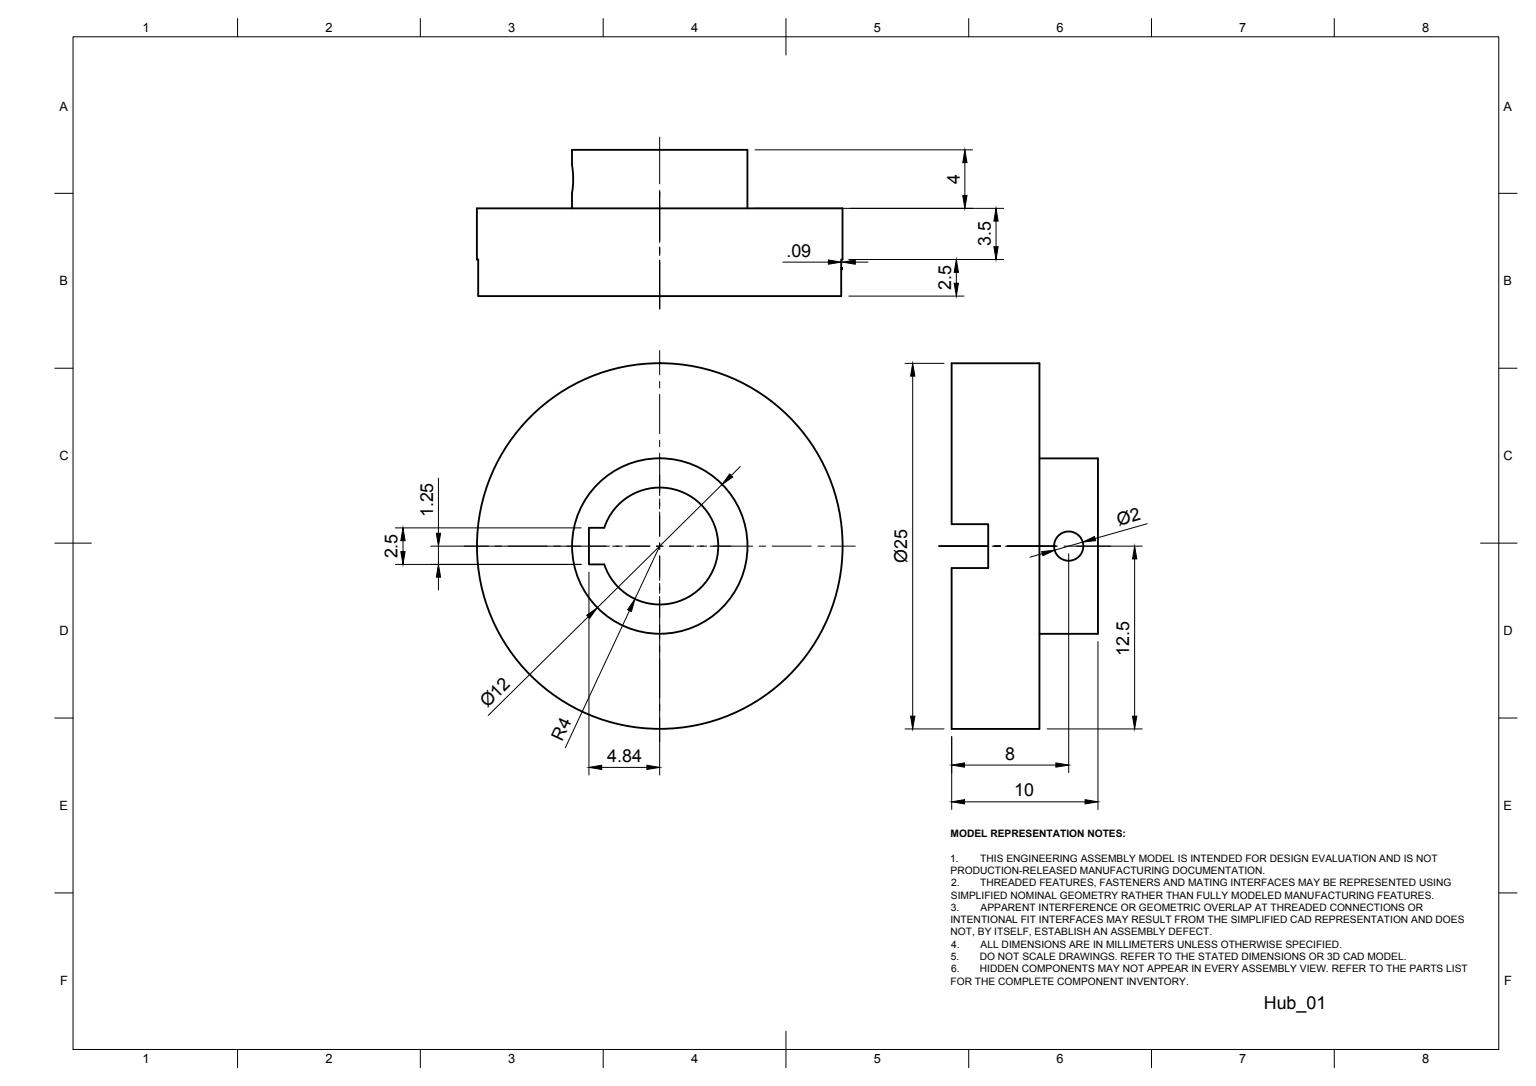
ISO-10303-21;
HEADER;
/* Generated by software containing ST-Developer
 * from STEP Tools, Inc. (www.steptools.com) 
 */

FILE_DESCRIPTION(
/* description */ (''),
/* implementation_level */ '2;1');

FILE_NAME(
/* name */ 'Hub_01.step',
/* time_stamp */ '2026-10-05T22:24:12-07:00',
/* author */ (''),
/* organization */ (''),
/* preprocessor_version */ 'ST-DEVELOPER v20.2',
/* originating_system */ 'Autodesk Translation Framework v15.15.0.0',
/* authorisation */ '');

FILE_SCHEMA (('AUTOMOTIVE_DESIGN { 1 0 10303 214 3 1 1 }'));
ENDSEC;

DATA;
#10=MECHANICAL_DESIGN_GEOMETRIC_PRESENTATION_REPRESENTATION('',(#53),#2116);
#39=SHAPE_REPRESENTATION_RELATIONSHIP('SRR','None',#2145,#46);
#46=ADVANCED_BREP_SHAPE_REPRESENTATION('',(#60),#2109);
#53=STYLED_ITEM('',(#2189),#60);
#60=MANIFOLD_SOLID_BREP('Body1',#1147);
#67=FACE_BOUND('',#201,.T.);
#68=FACE_BOUND('',#211,.T.);
#69=FACE_BOUND('',#213,.T.);
#70=FACE_BOUND('',#215,.T.);
#75=PLANE('',#1236);
#76=PLANE('',#1237);
#77=PLANE('',#1238);
#78=PLANE('',#1239);
#79=PLANE('',#1243);
#80=PLANE('',#1244);
#81=PLANE('',#1245);
#82=PLANE('',#1248);
#83=PLANE('',#1250);
#84=PLANE('',#1256);
#85=PLANE('',#1257);
#131=FACE_OUTER_BOUND('',#198,.T.);
#132=FACE_OUTER_BOUND('',#199,.T.);
#133=FACE_OUTER_BOUND('',#200,.T.);
#134=FACE_OUTER_BOUND('',#202,.T.);
#135=FACE_OUTER_BOUND('',#203,.T.);
#136=FACE_OUTER_BOUND('',#204,.T.);
#137=FACE_OUTER_BOUND('',#205,.T.);
#138=FACE_OUTER_BOUND('',#206,.T.);
#139=FACE_OUTER_BOUND('',#207,.T.);
#140=FACE_OUTER_BOUND('',#208,.T.);
#141=FACE_OUTER_BOUND('',#209,.T.);
#142=FACE_OUTER_BOUND('',#210,.T.);
#143=FACE_OUTER_BOUND('',#212,.T.);
#144=FACE_OUTER_BOUND('',#214,.T.);
#145=FACE_OUTER_BOUND('',#216,.T.);
#198=EDGE_LOOP('',(#773,#774,#775,#776));
#199=EDGE_LOOP('',(#777,#778,#779,#780));
#200=EDGE_LOOP('',(#781,#782,#783,#784));
#201=EDGE_LOOP('',(#785));
#202=EDGE_LOOP('',(#786,#787,#788,#789));
#203=EDGE_LOOP('',(#790,#791,#792,#793));
#204=EDGE_LOOP('',(#794,#795,#796,#797));
#205=EDGE_LOOP('',(#798,#799,#800,#801));
#206=EDGE_LOOP('',(#802,#803,#804,#805));
#207=EDGE_LOOP('',(#806,#807,#808,#809));
#208=EDGE_LOOP('',(#810,#811));
#209=EDGE_LOOP('',(#812,#813,#814));
#210=EDGE_LOOP('',(#815,#816,#817,#818));
#211=EDGE_LOOP('',(#819));
#212=EDGE_LOOP('',(#820));
#213=EDGE_LOOP('',(#821,#822,#823,#824));
#214=EDGE_LOOP('',(#825));
#215=EDGE_LOOP('',(#826));
#216=EDGE_LOOP('',(#827,#828,#829,#830,#831,#832,#833,#834,#835,#836,#837,
#838));
#273=B_SPLINE_CURVE_WITH_KNOTS('',3,(#1710,#1711,#1712,#1713,#1714,#1715,
#1716,#1717,#1718,#1719,#1720,#1721,#1722,#1723,#1724,#1725,#1726,#1727,
#1728,#1729,#1730,#1731,#1732,#1733,#1734,#1735,#1736,#1737,#1738,#1739,
#1740,#1741,#1742,#1743),.UNSPECIFIED.,.T.,.F.,(4,2,2,2,2,2,2,2,2,2,2,2,
2,2,2,2,4),(0.,0.0377449625945589,0.0754899251891177,0.113233879657539,
0.150977834125959,0.18872178859438,0.226465743062801,0.26421070565736,0.301955668251919,
0.339700630846477,0.377445593441036,0.415189547909457,0.452933502377878,
0.490677456846299,0.52842141131472,0.566166373909278,0.603911336503837),
 .UNSPECIFIED.);
#276=LINE('',#1709,#381);
#277=LINE('',#1747,#382);
#278=LINE('',#1749,#383);
#279=LINE('',#1751,#384);
#280=LINE('',#1752,#385);
#281=LINE('',#1755,#386);
#282=LINE('',#1757,#387);
#283=LINE('',#1758,#388);
#284=LINE('',#1761,#389);
#285=LINE('',#1763,#390);
#286=LINE('',#1764,#391);
#287=LINE('',#1772,#392);
#288=LINE('',#1774,#393);
#289=LINE('',#1776,#394);
#290=LINE('',#1777,#395);
#291=LINE('',#1781,#396);
#292=LINE('',#1783,#397);
#293=LINE('',#1785,#398);
#294=LINE('',#1786,#399);
#295=LINE('',#1800,#400);
#296=LINE('',#1807,#401);
#381=VECTOR('',#1362,1.);
#382=VECTOR('',#1365,10.);
#383=VECTOR('',#1366,10.);
#384=VECTOR('',#1367,10.);
#385=VECTOR('',#1368,10.);
#386=VECTOR('',#1371,10.);
#387=VECTOR('',#1372,10.);
#388=VECTOR('',#1373,10.);
#389=VECTOR('',#1376,10.);
#390=VECTOR('',#1377,10.);
#391=VECTOR('',#1378,10.);
#392=VECTOR('',#1389,10.);
#393=VECTOR('',#1390,10.);
#394=VECTOR('',#1391,10.);
#395=VECTOR('',#1392,10.);
#396=VECTOR('',#1395,10.);
#397=VECTOR('',#1396,10.);
#398=VECTOR('',#1397,10.);
#399=VECTOR('',#1398,10.);
#400=VECTOR('',#1419,6.);
#401=VECTOR('',#1430,12.5);
#486=CIRCLE('',#1235,1.);
#487=CIRCLE('',#1240,4.);
#488=CIRCLE('',#1242,4.);
#489=CIRCLE('',#1246,12.5);
#490=CIRCLE('',#1247,12.5);
#491=CIRCLE('',#1249,12.5);
#492=CIRCLE('',#1251,12.5);
#493=CIRCLE('',#1252,12.5);
#494=CIRCLE('',#1254,6.);
#495=CIRCLE('',#1255,6.);
#496=CIRCLE('',#1258,12.5);
#526=VERTEX_POINT('',#1706);
#527=VERTEX_POINT('',#1708);
#528=VERTEX_POINT('',#1745);
#529=VERTEX_POINT('',#1746);
#530=VERTEX_POINT('',#1748);
#531=VERTEX_POINT('',#1750);
#532=VERTEX_POINT('',#1754);
#533=VERTEX_POINT('',#1756);
#534=VERTEX_POINT('',#1760);
#535=VERTEX_POINT('',#1762);
#536=VERTEX_POINT('',#1770);
#537=VERTEX_POINT('',#1771);
#538=VERTEX_POINT('',#1773);
#539=VERTEX_POINT('',#1775);
#540=VERTEX_POINT('',#1779);
#541=VERTEX_POINT('',#1780);
#542=VERTEX_POINT('',#1782);
#543=VERTEX_POINT('',#1784);
#544=VERTEX_POINT('',#1793);
#545=VERTEX_POINT('',#1797);
#546=VERTEX_POINT('',#1799);
#547=VERTEX_POINT('',#1804);
#625=EDGE_CURVE('',#526,#526,#486,.T.);
#626=EDGE_CURVE('',#526,#527,#276,.T.);
#627=EDGE_CURVE('',#527,#527,#273,.T.);
#628=EDGE_CURVE('',#528,#529,#277,.T.);
#629=EDGE_CURVE('',#530,#528,#278,.T.);
#630=EDGE_CURVE('',#530,#531,#279,.T.);
#631=EDGE_CURVE('',#529,#531,#280,.T.);
#632=EDGE_CURVE('',#532,#528,#281,.T.);
#633=EDGE_CURVE('',#533,#532,#282,.T.);
#634=EDGE_CURVE('',#533,#530,#283,.T.);
#635=EDGE_CURVE('',#534,#532,#284,.T.);
#636=EDGE_CURVE('',#535,#534,#285,.T.);
#637=EDGE_CURVE('',#533,#535,#286,.T.);
#638=EDGE_CURVE('',#535,#531,#487,.T.);
#639=EDGE_CURVE('',#529,#534,#488,.T.);
#640=EDGE_CURVE('',#536,#537,#287,.T.);
#641=EDGE_CURVE('',#538,#536,#288,.T.);
#642=EDGE_CURVE('',#538,#539,#289,.T.);
#643=EDGE_CURVE('',#537,#539,#290,.T.);
#644=EDGE_CURVE('',#540,#541,#291,.T.);
#645=EDGE_CURVE('',#542,#540,#292,.T.);
#646=EDGE_CURVE('',#542,#543,#293,.T.);
#647=EDGE_CURVE('',#541,#543,#294,.T.);
#648=EDGE_CURVE('',#539,#542,#489,.T.);
#649=EDGE_CURVE('',#543,#538,#490,.T.);
#650=EDGE_CURVE('',#541,#540,#491,.T.);
#651=EDGE_CURVE('',#537,#544,#492,.T.);
#652=EDGE_CURVE('',#544,#536,#493,.T.);
#653=EDGE_CURVE('',#545,#545,#494,.T.);
#654=EDGE_CURVE('',#545,#546,#295,.T.);
#655=EDGE_CURVE('',#546,#546,#495,.T.);
#656=EDGE_CURVE('',#547,#547,#496,.T.);
#657=EDGE_CURVE('',#547,#544,#296,.T.);
#773=ORIENTED_EDGE('',*,*,#625,.F.);
#774=ORIENTED_EDGE('',*,*,#626,.T.);
#775=ORIENTED_EDGE('',*,*,#627,.F.);
#776=ORIENTED_EDGE('',*,*,#626,.F.);
#777=ORIENTED_EDGE('',*,*,#628,.F.);
#778=ORIENTED_EDGE('',*,*,#629,.F.);
#779=ORIENTED_EDGE('',*,*,#630,.T.);
#780=ORIENTED_EDGE('',*,*,#631,.F.);
#781=ORIENTED_EDGE('',*,*,#632,.F.);
#782=ORIENTED_EDGE('',*,*,#633,.F.);
#783=ORIENTED_EDGE('',*,*,#634,.T.);
#784=ORIENTED_EDGE('',*,*,#629,.T.);
#785=ORIENTED_EDGE('',*,*,#625,.T.);
#786=ORIENTED_EDGE('',*,*,#635,.F.);
#787=ORIENTED_EDGE('',*,*,#636,.F.);
#788=ORIENTED_EDGE('',*,*,#637,.F.);
#789=ORIENTED_EDGE('',*,*,#633,.T.);
#790=ORIENTED_EDGE('',*,*,#638,.T.);
#791=ORIENTED_EDGE('',*,*,#630,.F.);
#792=ORIENTED_EDGE('',*,*,#634,.F.);
#793=ORIENTED_EDGE('',*,*,#637,.T.);
#794=ORIENTED_EDGE('',*,*,#631,.T.);
#795=ORIENTED_EDGE('',*,*,#638,.F.);
#796=ORIENTED_EDGE('',*,*,#636,.T.);
#797=ORIENTED_EDGE('',*,*,#639,.F.);
#798=ORIENTED_EDGE('',*,*,#640,.F.);
#799=ORIENTED_EDGE('',*,*,#641,.F.);
#800=ORIENTED_EDGE('',*,*,#642,.T.);
#801=ORIENTED_EDGE('',*,*,#643,.F.);
#802=ORIENTED_EDGE('',*,*,#644,.F.);
#803=ORIENTED_EDGE('',*,*,#645,.F.);
#804=ORIENTED_EDGE('',*,*,#646,.T.);
#805=ORIENTED_EDGE('',*,*,#647,.F.);
#806=ORIENTED_EDGE('',*,*,#648,.F.);
#807=ORIENTED_EDGE('',*,*,#642,.F.);
#808=ORIENTED_EDGE('',*,*,#649,.F.);
#809=ORIENTED_EDGE('',*,*,#646,.F.);
#810=ORIENTED_EDGE('',*,*,#644,.T.);
#811=ORIENTED_EDGE('',*,*,#650,.T.);
#812=ORIENTED_EDGE('',*,*,#640,.T.);
#813=ORIENTED_EDGE('',*,*,#651,.T.);
#814=ORIENTED_EDGE('',*,*,#652,.T.);
#815=ORIENTED_EDGE('',*,*,#653,.F.);
#816=ORIENTED_EDGE('',*,*,#654,.T.);
#817=ORIENTED_EDGE('',*,*,#655,.F.);
#818=ORIENTED_EDGE('',*,*,#654,.F.);
#819=ORIENTED_EDGE('',*,*,#627,.T.);
#820=ORIENTED_EDGE('',*,*,#653,.T.);
#821=ORIENTED_EDGE('',*,*,#628,.T.);
#822=ORIENTED_EDGE('',*,*,#639,.T.);
#823=ORIENTED_EDGE('',*,*,#635,.T.);
#824=ORIENTED_EDGE('',*,*,#632,.T.);
#825=ORIENTED_EDGE('',*,*,#656,.T.);
#826=ORIENTED_EDGE('',*,*,#655,.T.);
#827=ORIENTED_EDGE('',*,*,#656,.F.);
#828=ORIENTED_EDGE('',*,*,#657,.T.);
#829=ORIENTED_EDGE('',*,*,#651,.F.);
#830=ORIENTED_EDGE('',*,*,#643,.T.);
#831=ORIENTED_EDGE('',*,*,#648,.T.);
#832=ORIENTED_EDGE('',*,*,#645,.T.);
#833=ORIENTED_EDGE('',*,*,#650,.F.);
#834=ORIENTED_EDGE('',*,*,#647,.T.);
#835=ORIENTED_EDGE('',*,*,#649,.T.);
#836=ORIENTED_EDGE('',*,*,#641,.T.);
#837=ORIENTED_EDGE('',*,*,#652,.F.);
#838=ORIENTED_EDGE('',*,*,#657,.F.);
#1069=CYLINDRICAL_SURFACE('',#1234,1.);
#1070=CYLINDRICAL_SURFACE('',#1241,4.);
#1071=CYLINDRICAL_SURFACE('',#1253,6.);
#1072=CYLINDRICAL_SURFACE('',#1259,12.5);
#1080=ADVANCED_FACE('',(#131),#1069,.F.);
#1081=ADVANCED_FACE('',(#132),#75,.F.);
#1082=ADVANCED_FACE('',(#133,#67),#76,.F.);
#1083=ADVANCED_FACE('',(#134),#77,.F.);
#1084=ADVANCED_FACE('',(#135),#78,.F.);
#1085=ADVANCED_FACE('',(#136),#1070,.F.);
#1086=ADVANCED_FACE('',(#137),#79,.F.);
#1087=ADVANCED_FACE('',(#138),#80,.F.);
#1088=ADVANCED_FACE('',(#139),#81,.T.);
#1089=ADVANCED_FACE('',(#140),#82,.T.);
#1090=ADVANCED_FACE('',(#141),#83,.T.);
#1091=ADVANCED_FACE('',(#142,#68),#1071,.T.);
#1092=ADVANCED_FACE('',(#143,#69),#84,.T.);
#1093=ADVANCED_FACE('',(#144,#70),#85,.F.);
#1094=ADVANCED_FACE('',(#145),#1072,.T.);
#1147=CLOSED_SHELL('',(#1080,#1081,#1082,#1083,#1084,#1085,#1086,#1087,
#1088,#1089,#1090,#1091,#1092,#1093,#1094));
#1233=AXIS2_PLACEMENT_3D('',#1704,#1356,#1357);
#1234=AXIS2_PLACEMENT_3D('',#1705,#1358,#1359);
#1235=AXIS2_PLACEMENT_3D('',#1707,#1360,#1361);
#1236=AXIS2_PLACEMENT_3D('',#1744,#1363,#1364);
#1237=AXIS2_PLACEMENT_3D('',#1753,#1369,#1370);
#1238=AXIS2_PLACEMENT_3D('',#1759,#1374,#1375);
#1239=AXIS2_PLACEMENT_3D('',#1765,#1379,#1380);
#1240=AXIS2_PLACEMENT_3D('',#1766,#1381,#1382);
#1241=AXIS2_PLACEMENT_3D('',#1767,#1383,#1384);
#1242=AXIS2_PLACEMENT_3D('',#1768,#1385,#1386);
#1243=AXIS2_PLACEMENT_3D('',#1769,#1387,#1388);
#1244=AXIS2_PLACEMENT_3D('',#1778,#1393,#1394);
#1245=AXIS2_PLACEMENT_3D('',#1787,#1399,#1400);
#1246=AXIS2_PLACEMENT_3D('',#1788,#1401,#1402);
#1247=AXIS2_PLACEMENT_3D('',#1789,#1403,#1404);
#1248=AXIS2_PLACEMENT_3D('',#1790,#1405,#1406);
#1249=AXIS2_PLACEMENT_3D('',#1791,#1407,#1408);
#1250=AXIS2_PLACEMENT_3D('',#1792,#1409,#1410);
#1251=AXIS2_PLACEMENT_3D('',#1794,#1411,#1412);
#1252=AXIS2_PLACEMENT_3D('',#1795,#1413,#1414);
#1253=AXIS2_PLACEMENT_3D('',#1796,#1415,#1416);
#1254=AXIS2_PLACEMENT_3D('',#1798,#1417,#1418);
#1255=AXIS2_PLACEMENT_3D('',#1801,#1420,#1421);
#1256=AXIS2_PLACEMENT_3D('',#1802,#1422,#1423);
#1257=AXIS2_PLACEMENT_3D('',#1803,#1424,#1425);
#1258=AXIS2_PLACEMENT_3D('',#1805,#1426,#1427);
#1259=AXIS2_PLACEMENT_3D('',#1806,#1428,#1429);
#1356=DIRECTION('axis',(0.,0.,1.));
#1357=DIRECTION('refdir',(1.,0.,0.));
#1358=DIRECTION('center_axis',(0.,0.,1.));
#1359=DIRECTION('ref_axis',(1.,0.,0.));
#1360=DIRECTION('center_axis',(0.,0.,1.));
#1361=DIRECTION('ref_axis',(1.,0.,0.));
#1362=DIRECTION('',(0.,0.,1.));
#1363=DIRECTION('center_axis',(1.,0.,0.));
#1364=DIRECTION('ref_axis',(0.,0.,1.));
#1365=DIRECTION('',(0.,0.,-1.));
#1366=DIRECTION('',(0.,-1.,0.));
#1367=DIRECTION('',(0.,0.,-1.));
#1368=DIRECTION('',(0.,1.,0.));
#1369=DIRECTION('center_axis',(0.,0.,1.));
#1370=DIRECTION('ref_axis',(-1.,0.,0.));
#1371=DIRECTION('',(1.,0.,0.));
#1372=DIRECTION('',(0.,-1.,0.));
#1373=DIRECTION('',(1.,0.,0.));
#1374=DIRECTION('center_axis',(-1.,0.,0.));
#1375=DIRECTION('ref_axis',(0.,0.,-1.));
#1376=DIRECTION('',(0.,0.,1.));
#1377=DIRECTION('',(0.,-1.,0.));
#1378=DIRECTION('',(0.,0.,-1.));
#1379=DIRECTION('center_axis',(0.,1.,0.));
#1380=DIRECTION('ref_axis',(1.,0.,0.));
#1381=DIRECTION('center_axis',(0.,-1.,0.));
#1382=DIRECTION('ref_axis',(1.,0.,0.));
#1383=DIRECTION('center_axis',(0.,-1.,0.));
#1384=DIRECTION('ref_axis',(6.12323399573677E-17,0.,-1.));
#1385=DIRECTION('center_axis',(0.,1.,0.));
#1386=DIRECTION('ref_axis',(1.,0.,0.));
#1387=DIRECTION('center_axis',(-1.,0.,0.));
#1388=DIRECTION('ref_axis',(0.,0.,-1.));
#1389=DIRECTION('',(0.,0.,-1.));
#1390=DIRECTION('',(0.,1.,0.));
#1391=DIRECTION('',(0.,0.,-1.));
#1392=DIRECTION('',(0.,-1.,0.));
#1393=DIRECTION('center_axis',(1.,0.,0.));
#1394=DIRECTION('ref_axis',(0.,0.,1.));
#1395=DIRECTION('',(0.,0.,1.));
#1396=DIRECTION('',(0.,1.,0.));
#1397=DIRECTION('',(0.,0.,1.));
#1398=DIRECTION('',(0.,-1.,0.));
#1399=DIRECTION('center_axis',(0.,1.,0.));
#1400=DIRECTION('ref_axis',(-1.,0.,0.));
#1401=DIRECTION('center_axis',(0.,-1.,0.));
#1402=DIRECTION('ref_axis',(1.,0.,0.));
#1403=DIRECTION('center_axis',(0.,-1.,0.));
#1404=DIRECTION('ref_axis',(1.,0.,0.));
#1405=DIRECTION('center_axis',(0.,1.,0.));
#1406=DIRECTION('ref_axis',(1.,0.,0.));
#1407=DIRECTION('center_axis',(0.,1.,0.));
#1408=DIRECTION('ref_axis',(1.,0.,0.));
#1409=DIRECTION('center_axis',(0.,1.,0.));
#1410=DIRECTION('ref_axis',(1.,0.,0.));
#1411=DIRECTION('center_axis',(0.,1.,0.));
#1412=DIRECTION('ref_axis',(1.,0.,0.));
#1413=DIRECTION('center_axis',(0.,1.,0.));
#1414=DIRECTION('ref_axis',(1.,0.,0.));
#1415=DIRECTION('center_axis',(0.,-1.,0.));
#1416=DIRECTION('ref_axis',(1.,0.,0.));
#1417=DIRECTION('center_axis',(0.,-1.,0.));
#1418=DIRECTION('ref_axis',(1.,0.,0.));
#1419=DIRECTION('',(0.,1.,0.));
#1420=DIRECTION('center_axis',(0.,1.,0.));
#1421=DIRECTION('ref_axis',(1.,0.,0.));
#1422=DIRECTION('center_axis',(0.,-1.,0.));
#1423=DIRECTION('ref_axis',(1.,0.,0.));
#1424=DIRECTION('center_axis',(0.,1.,0.));
#1425=DIRECTION('ref_axis',(1.,0.,0.));
#1426=DIRECTION('center_axis',(0.,-1.,0.));
#1427=DIRECTION('ref_axis',(1.,0.,0.));
#1428=DIRECTION('center_axis',(0.,-1.,0.));
#1429=DIRECTION('ref_axis',(1.,0.,0.));
#1430=DIRECTION('',(0.,1.,0.));
#1704=CARTESIAN_POINT('',(0.,0.,0.));
#1705=CARTESIAN_POINT('Origin',(0.,-8.,0.));
#1706=CARTESIAN_POINT('',(-1.,-8.,4.84122918275927));
#1707=CARTESIAN_POINT('Origin',(0.,-8.,4.84122918275927));
#1708=CARTESIAN_POINT('',(-1.,-8.,5.91607978309962));
#1709=CARTESIAN_POINT('',(-1.,-8.,0.));
#1710=CARTESIAN_POINT('Ctrl Pts',(-1.,-8.,5.91607978309962));
#1711=CARTESIAN_POINT('Ctrl Pts',(-1.,-7.87418345801814,5.91607978309962));
#1712=CARTESIAN_POINT('Ctrl Pts',(-0.974807371025508,-7.74014451903107,
5.92050853647266));
#1713=CARTESIAN_POINT('Ctrl Pts',(-0.872681546203438,-7.49383674704903,
5.93642128117897));
#1714=CARTESIAN_POINT('Ctrl Pts',(-0.795760896484534,-7.38154733411144,
5.94766633611059));
#1715=CARTESIAN_POINT('Ctrl Pts',(-0.61845503374177,-7.20424147136868,5.96870867068992));
#1716=CARTESIAN_POINT('Ctrl Pts',(-0.506164604242066,-7.12731896437637,
5.97988517961729));
#1717=CARTESIAN_POINT('Ctrl Pts',(-0.25985334006496,-7.0251917910001,5.99564055034545));
#1718=CARTESIAN_POINT('Ctrl Pts',(-0.125813181561402,-7.,6.));
#1719=CARTESIAN_POINT('Ctrl Pts',(0.125813181561403,-7.,6.));
#1720=CARTESIAN_POINT('Ctrl Pts',(0.259853340064961,-7.0251917910001,5.99564055034545));
#1721=CARTESIAN_POINT('Ctrl Pts',(0.506164604242067,-7.12731896437637,5.97988517961729));
#1722=CARTESIAN_POINT('Ctrl Pts',(0.618455033741771,-7.20424147136868,5.96870867068992));
#1723=CARTESIAN_POINT('Ctrl Pts',(0.795760896484535,-7.38154733411144,5.94766633611059));
#1724=CARTESIAN_POINT('Ctrl Pts',(0.872681546203439,-7.49383674704903,5.93642128117897));
#1725=CARTESIAN_POINT('Ctrl Pts',(0.974807371025509,-7.74014451903108,5.92050853647266));
#1726=CARTESIAN_POINT('Ctrl Pts',(1.,-7.87418345801814,5.91607978309962));
#1727=CARTESIAN_POINT('Ctrl Pts',(1.,-8.12581654198186,5.91607978309962));
#1728=CARTESIAN_POINT('Ctrl Pts',(0.974807371025508,-8.25985548096893,5.92050853647266));
#1729=CARTESIAN_POINT('Ctrl Pts',(0.872681546203439,-8.50616325295097,5.93642128117897));
#1730=CARTESIAN_POINT('Ctrl Pts',(0.795760896484535,-8.61845266588856,5.94766633611059));
#1731=CARTESIAN_POINT('Ctrl Pts',(0.618455033741771,-8.79575852863132,5.96870867068992));
#1732=CARTESIAN_POINT('Ctrl Pts',(0.506164604242067,-8.87268103562363,5.97988517961729));
#1733=CARTESIAN_POINT('Ctrl Pts',(0.25985334006496,-8.97480820899991,5.99564055034545));
#1734=CARTESIAN_POINT('Ctrl Pts',(0.125813181561403,-9.,6.));
#1735=CARTESIAN_POINT('Ctrl Pts',(-0.125813181561403,-9.,6.));
#1736=CARTESIAN_POINT('Ctrl Pts',(-0.25985334006496,-8.97480820899991,5.99564055034545));
#1737=CARTESIAN_POINT('Ctrl Pts',(-0.506164604242066,-8.87268103562363,
5.97988517961729));
#1738=CARTESIAN_POINT('Ctrl Pts',(-0.618455033741771,-8.79575852863132,
5.96870867068992));
#1739=CARTESIAN_POINT('Ctrl Pts',(-0.795760896484535,-8.61845266588856,
5.94766633611059));
#1740=CARTESIAN_POINT('Ctrl Pts',(-0.872681546203439,-8.50616325295097,
5.93642128117897));
#1741=CARTESIAN_POINT('Ctrl Pts',(-0.974807371025509,-8.25985548096893,
5.92050853647266));
#1742=CARTESIAN_POINT('Ctrl Pts',(-1.,-8.12581654198186,5.91607978309962));
#1743=CARTESIAN_POINT('Ctrl Pts',(-1.,-8.,5.91607978309962));
#1744=CARTESIAN_POINT('Origin',(1.25,-6.,3.29967103839267));
#1745=CARTESIAN_POINT('',(1.25,-10.,4.84122918275927));
#1746=CARTESIAN_POINT('',(1.25,-10.,3.79967103839267));
#1747=CARTESIAN_POINT('',(1.25,-10.,1.64983551919633));
#1748=CARTESIAN_POINT('',(1.25,-6.,4.84122918275927));
#1749=CARTESIAN_POINT('',(1.25,-6.,4.84122918275927));
#1750=CARTESIAN_POINT('',(1.25,-6.,3.79967103839267));
#1751=CARTESIAN_POINT('',(1.25,-6.,6.32461990770089));
#1752=CARTESIAN_POINT('',(1.25,-6.,3.79967103839267));
#1753=CARTESIAN_POINT('Origin',(1.25,-6.,4.84122918275927));
#1754=CARTESIAN_POINT('',(-1.25,-10.,4.84122918275927));
#1755=CARTESIAN_POINT('',(0.625,-10.,4.84122918275927));
#1756=CARTESIAN_POINT('',(-1.25,-6.,4.84122918275927));
#1757=CARTESIAN_POINT('',(-1.25,-6.,4.84122918275927));
#1758=CARTESIAN_POINT('',(-1.25,-6.,4.84122918275927));
#1759=CARTESIAN_POINT('Origin',(-1.25,-6.,4.84122918275927));
#1760=CARTESIAN_POINT('',(-1.25,-10.,3.79967103839267));
#1761=CARTESIAN_POINT('',(-1.25,-10.,2.42061459137964));
#1762=CARTESIAN_POINT('',(-1.25,-6.,3.79967103839267));
#1763=CARTESIAN_POINT('',(-1.25,-6.,3.79967103839267));
#1764=CARTESIAN_POINT('',(-1.25,-6.,3.79967103839267));
#1765=CARTESIAN_POINT('Origin',(0.,-6.,0.));
#1766=CARTESIAN_POINT('Origin',(0.,-6.,0.));
#1767=CARTESIAN_POINT('Origin',(0.,-6.,0.));
#1768=CARTESIAN_POINT('Origin',(0.,-10.,0.));
#1769=CARTESIAN_POINT('Origin',(-1.5,0.,12.4096736459909));
#1770=CARTESIAN_POINT('',(-1.5,0.,12.4096736459909));
#1771=CARTESIAN_POINT('',(-1.5,0.,-12.4096736459909));
#1772=CARTESIAN_POINT('',(-1.5,0.,6.20483682299543));
#1773=CARTESIAN_POINT('',(-1.5,-2.5,12.4096736459909));
#1774=CARTESIAN_POINT('',(-1.5,0.,12.4096736459909));
#1775=CARTESIAN_POINT('',(-1.5,-2.5,-12.4096736459909));
#1776=CARTESIAN_POINT('',(-1.5,-2.5,15.2595947063511));
#1777=CARTESIAN_POINT('',(-1.5,0.,-12.4096736459909));
#1778=CARTESIAN_POINT('Origin',(1.5,0.,-12.4096736459909));
#1779=CARTESIAN_POINT('',(1.5,0.,-12.4096736459909));
#1780=CARTESIAN_POINT('',(1.5,0.,12.4096736459909));
#1781=CARTESIAN_POINT('',(1.5,0.,-6.20483682299543));
#1782=CARTESIAN_POINT('',(1.5,-2.5,-12.4096736459909));
#1783=CARTESIAN_POINT('',(1.5,0.,-12.4096736459909));
#1784=CARTESIAN_POINT('',(1.5,-2.5,12.4096736459909));
#1785=CARTESIAN_POINT('',(1.5,-2.5,-15.2595947063511));
#1786=CARTESIAN_POINT('',(1.5,0.,12.4096736459909));
#1787=CARTESIAN_POINT('Origin',(2.77555756156289E-16,-2.5,0.));
#1788=CARTESIAN_POINT('Origin',(0.,-2.5,0.));
#1789=CARTESIAN_POINT('Origin',(0.,-2.5,0.));
#1790=CARTESIAN_POINT('Origin',(0.,0.,0.));
#1791=CARTESIAN_POINT('Origin',(0.,0.,0.));
#1792=CARTESIAN_POINT('Origin',(0.,0.,0.));
#1793=CARTESIAN_POINT('',(-12.5,0.,-1.53080849893419E-15));
#1794=CARTESIAN_POINT('Origin',(0.,0.,0.));
#1795=CARTESIAN_POINT('Origin',(0.,0.,0.));
#1796=CARTESIAN_POINT('Origin',(0.,-6.,0.));
#1797=CARTESIAN_POINT('',(-6.,-10.,-7.34788079488412E-16));
#1798=CARTESIAN_POINT('Origin',(0.,-10.,0.));
#1799=CARTESIAN_POINT('',(-6.,-6.,-7.34788079488412E-16));
#1800=CARTESIAN_POINT('',(-6.,-6.,-7.34788079488412E-16));
#1801=CARTESIAN_POINT('Origin',(0.,-6.,0.));
#1802=CARTESIAN_POINT('Origin',(0.,-10.,0.));
#1803=CARTESIAN_POINT('Origin',(0.,-6.,0.));
#1804=CARTESIAN_POINT('',(-12.5,-6.,1.53080849893419E-15));
#1805=CARTESIAN_POINT('Origin',(0.,-6.,0.));
#1806=CARTESIAN_POINT('Origin',(0.,0.,0.));
#1807=CARTESIAN_POINT('',(-12.5,0.,-1.53080849893419E-15));
#2100=UNCERTAINTY_MEASURE_WITH_UNIT(LENGTH_MEASURE(0.01),#2117,
'DISTANCE_ACCURACY_VALUE',
'Maximum model space distance between geometric entities at asserted c
onnectivities');
#2107=UNCERTAINTY_MEASURE_WITH_UNIT(LENGTH_MEASURE(0.01),#2117,
'DISTANCE_ACCURACY_VALUE',
'Maximum model space distance between geometric entities at asserted c
onnectivities');
#2109=(
GEOMETRIC_REPRESENTATION_CONTEXT(3)
GLOBAL_UNCERTAINTY_ASSIGNED_CONTEXT((#2100))
GLOBAL_UNIT_ASSIGNED_CONTEXT((#2117,#2119,#2120))
REPRESENTATION_CONTEXT('','3D')
);
#2116=(
GEOMETRIC_REPRESENTATION_CONTEXT(3)
GLOBAL_UNCERTAINTY_ASSIGNED_CONTEXT((#2107))
GLOBAL_UNIT_ASSIGNED_CONTEXT((#2117,#2119,#2120))
REPRESENTATION_CONTEXT('','3D')
);
#2117=(
LENGTH_UNIT()
NAMED_UNIT(*)
SI_UNIT(.MILLI.,.METRE.)
);
#2119=(
NAMED_UNIT(*)
PLANE_ANGLE_UNIT()
SI_UNIT($,.RADIAN.)
);
#2120=(
NAMED_UNIT(*)
SI_UNIT($,.STERADIAN.)
SOLID_ANGLE_UNIT()
);
#2122=SHAPE_DEFINITION_REPRESENTATION(#2130,#2145);
#2130=PRODUCT_DEFINITION_SHAPE('',$,#2154);
#2145=SHAPE_REPRESENTATION('',(#1233),#2109);
#2152=PRODUCT_DEFINITION_CONTEXT('part definition',#2178,'design');
#2154=PRODUCT_DEFINITION('Hub_01','Hub_01',#2162,#2152);
#2162=PRODUCT_DEFINITION_FORMATION('',$,#2181);
#2178=APPLICATION_CONTEXT(
'Core Data for Automotive Mechanical Design Process');
#2179=PRODUCT_CONTEXT('part definition',#2178,'mechanical');
#2181=PRODUCT('Hub_01','Hub_01',$,(#2179));
#2189=PRESENTATION_STYLE_ASSIGNMENT((#2194));
#2194=SURFACE_STYLE_USAGE(.BOTH.,#2199);
#2199=SURFACE_SIDE_STYLE('',(#2204));
#2204=SURFACE_STYLE_FILL_AREA(#2209);
#2209=FILL_AREA_STYLE('Opaque(0,188,0)',(#2214));
#2214=FILL_AREA_STYLE_COLOUR('Opaque(0,188,0)',#2219);
#2219=COLOUR_RGB('Opaque(0,188,0)', 0.09019608, 0.27058824, 0.51372549);
ENDSEC;
END-ISO-10303-21;
